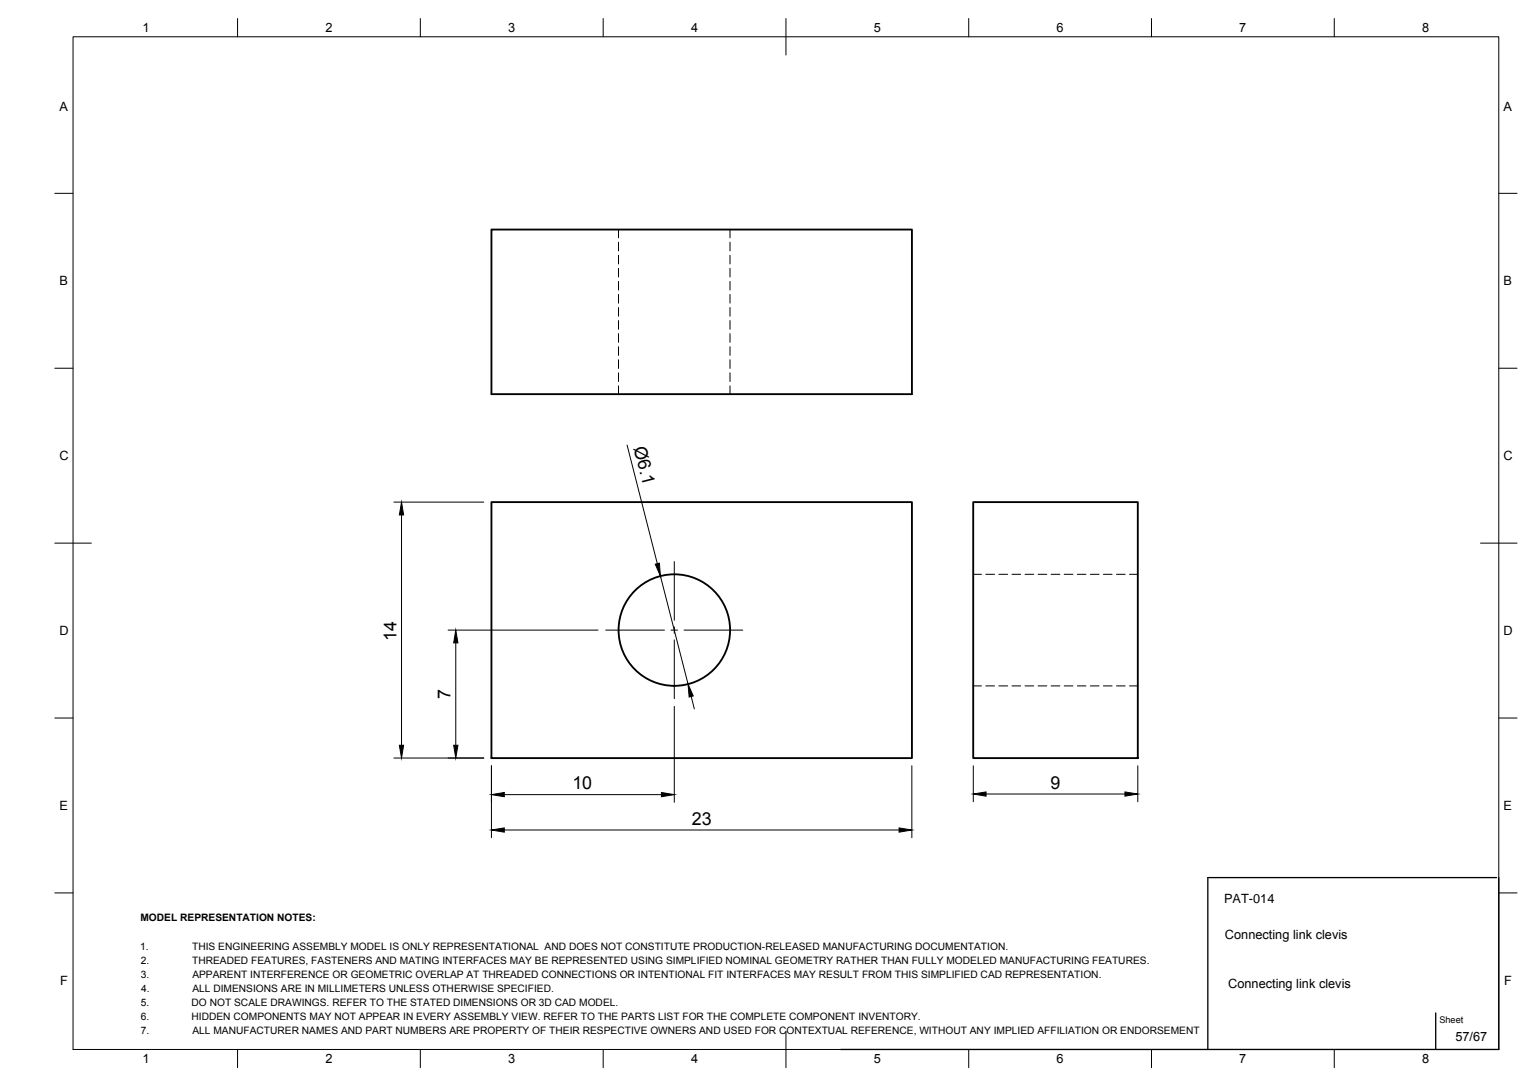
ISO-10303-21;
HEADER;
/* Generated by software containing ST-Developer
 * from STEP Tools, Inc. (www.steptools.com) 
 */

FILE_DESCRIPTION(
/* description */ ('Bin tilter linkage'),
/* implementation_level */ '2;1');

FILE_NAME(
/* name */ 'Connecting link clevis.step',
/* time_stamp */ '2026-10-28T03:26:24-07:00',
/* author */ (''),
/* organization */ (''),
/* preprocessor_version */ 'ST-DEVELOPER v20.2',
/* originating_system */ 'Autodesk Translation Framework v15.17.0.0',
/* authorisation */ '');

FILE_SCHEMA (('AUTOMOTIVE_DESIGN { 1 0 10303 214 3 1 1 }'));
ENDSEC;

DATA;
#10=MECHANICAL_DESIGN_GEOMETRIC_PRESENTATION_REPRESENTATION('',(#963),#23728);
#743=SHAPE_REPRESENTATION_RELATIONSHIP('SRR','None',#24212,#849);
#849=ADVANCED_BREP_SHAPE_REPRESENTATION('',(#1075),#23712);
#963=STYLED_ITEM('',(#24751),#1075);
#1075=MANIFOLD_SOLID_BREP('Body1',#12495);
#1462=FACE_BOUND('',#3732,.T.);
#1463=FACE_BOUND('',#3735,.T.);
#1834=PLANE('',#15279);
#1835=PLANE('',#15280);
#1836=PLANE('',#15281);
#1837=PLANE('',#15282);
#1838=PLANE('',#15283);
#1839=PLANE('',#15284);
#2578=FACE_OUTER_BOUND('',#3730,.T.);
#2579=FACE_OUTER_BOUND('',#3731,.T.);
#2580=FACE_OUTER_BOUND('',#3733,.T.);
#2581=FACE_OUTER_BOUND('',#3734,.T.);
#2582=FACE_OUTER_BOUND('',#3736,.T.);
#2583=FACE_OUTER_BOUND('',#3737,.T.);
#2584=FACE_OUTER_BOUND('',#3738,.T.);
#3730=EDGE_LOOP('',(#10955,#10956,#10957,#10958));
#3731=EDGE_LOOP('',(#10959,#10960,#10961,#10962));
#3732=EDGE_LOOP('',(#10963));
#3733=EDGE_LOOP('',(#10964,#10965,#10966,#10967));
#3734=EDGE_LOOP('',(#10968,#10969,#10970,#10971));
#3735=EDGE_LOOP('',(#10972));
#3736=EDGE_LOOP('',(#10973,#10974,#10975,#10976));
#3737=EDGE_LOOP('',(#10977,#10978,#10979,#10980));
#3738=EDGE_LOOP('',(#10981,#10982,#10983,#10984));
#4437=LINE('',#23111,#5112);
#4438=LINE('',#23116,#5113);
#4439=LINE('',#23118,#5114);
#4440=LINE('',#23120,#5115);
#4441=LINE('',#23121,#5116);
#4442=LINE('',#23124,#5117);
#4443=LINE('',#23126,#5118);
#4444=LINE('',#23127,#5119);
#4445=LINE('',#23130,#5120);
#4446=LINE('',#23132,#5121);
#4447=LINE('',#23133,#5122);
#4448=LINE('',#23135,#5123);
#4449=LINE('',#23136,#5124);
#5112=VECTOR('',#19266,0.305);
#5113=VECTOR('',#19271,1.);
#5114=VECTOR('',#19272,1.);
#5115=VECTOR('',#19273,1.);
#5116=VECTOR('',#19274,1.);
#5117=VECTOR('',#19277,1.);
#5118=VECTOR('',#19278,1.);
#5119=VECTOR('',#19279,1.);
#5120=VECTOR('',#19282,1.);
#5121=VECTOR('',#19283,1.);
#5122=VECTOR('',#19284,1.);
#5123=VECTOR('',#19287,1.);
#5124=VECTOR('',#19288,1.);
#5888=CIRCLE('',#15277,0.305);
#5889=CIRCLE('',#15278,0.305);
#6823=VERTEX_POINT('',#23108);
#6824=VERTEX_POINT('',#23110);
#6825=VERTEX_POINT('',#23114);
#6826=VERTEX_POINT('',#23115);
#6827=VERTEX_POINT('',#23117);
#6828=VERTEX_POINT('',#23119);
#6829=VERTEX_POINT('',#23123);
#6830=VERTEX_POINT('',#23125);
#6831=VERTEX_POINT('',#23129);
#6832=VERTEX_POINT('',#23131);
#8217=EDGE_CURVE('',#6823,#6823,#5888,.T.);
#8218=EDGE_CURVE('',#6823,#6824,#4437,.T.);
#8219=EDGE_CURVE('',#6824,#6824,#5889,.T.);
#8220=EDGE_CURVE('',#6825,#6826,#4438,.T.);
#8221=EDGE_CURVE('',#6826,#6827,#4439,.T.);
#8222=EDGE_CURVE('',#6828,#6827,#4440,.T.);
#8223=EDGE_CURVE('',#6825,#6828,#4441,.T.);
#8224=EDGE_CURVE('',#6829,#6825,#4442,.T.);
#8225=EDGE_CURVE('',#6830,#6828,#4443,.T.);
#8226=EDGE_CURVE('',#6829,#6830,#4444,.T.);
#8227=EDGE_CURVE('',#6831,#6829,#4445,.T.);
#8228=EDGE_CURVE('',#6832,#6830,#4446,.T.);
#8229=EDGE_CURVE('',#6831,#6832,#4447,.T.);
#8230=EDGE_CURVE('',#6826,#6831,#4448,.T.);
#8231=EDGE_CURVE('',#6827,#6832,#4449,.T.);
#10955=ORIENTED_EDGE('',*,*,#8217,.F.);
#10956=ORIENTED_EDGE('',*,*,#8218,.T.);
#10957=ORIENTED_EDGE('',*,*,#8219,.F.);
#10958=ORIENTED_EDGE('',*,*,#8218,.F.);
#10959=ORIENTED_EDGE('',*,*,#8220,.T.);
#10960=ORIENTED_EDGE('',*,*,#8221,.T.);
#10961=ORIENTED_EDGE('',*,*,#8222,.F.);
#10962=ORIENTED_EDGE('',*,*,#8223,.F.);
#10963=ORIENTED_EDGE('',*,*,#8219,.T.);
#10964=ORIENTED_EDGE('',*,*,#8224,.T.);
#10965=ORIENTED_EDGE('',*,*,#8223,.T.);
#10966=ORIENTED_EDGE('',*,*,#8225,.F.);
#10967=ORIENTED_EDGE('',*,*,#8226,.F.);
#10968=ORIENTED_EDGE('',*,*,#8227,.T.);
#10969=ORIENTED_EDGE('',*,*,#8226,.T.);
#10970=ORIENTED_EDGE('',*,*,#8228,.F.);
#10971=ORIENTED_EDGE('',*,*,#8229,.F.);
#10972=ORIENTED_EDGE('',*,*,#8217,.T.);
#10973=ORIENTED_EDGE('',*,*,#8230,.T.);
#10974=ORIENTED_EDGE('',*,*,#8229,.T.);
#10975=ORIENTED_EDGE('',*,*,#8231,.F.);
#10976=ORIENTED_EDGE('',*,*,#8221,.F.);
#10977=ORIENTED_EDGE('',*,*,#8231,.T.);
#10978=ORIENTED_EDGE('',*,*,#8228,.T.);
#10979=ORIENTED_EDGE('',*,*,#8225,.T.);
#10980=ORIENTED_EDGE('',*,*,#8222,.T.);
#10981=ORIENTED_EDGE('',*,*,#8230,.F.);
#10982=ORIENTED_EDGE('',*,*,#8220,.F.);
#10983=ORIENTED_EDGE('',*,*,#8224,.F.);
#10984=ORIENTED_EDGE('',*,*,#8227,.F.);
#11585=CYLINDRICAL_SURFACE('',#15276,0.305);
#12303=ADVANCED_FACE('',(#2578),#11585,.F.);
#12304=ADVANCED_FACE('',(#2579,#1462),#1834,.T.);
#12305=ADVANCED_FACE('',(#2580),#1835,.T.);
#12306=ADVANCED_FACE('',(#2581,#1463),#1836,.T.);
#12307=ADVANCED_FACE('',(#2582),#1837,.T.);
#12308=ADVANCED_FACE('',(#2583),#1838,.T.);
#12309=ADVANCED_FACE('',(#2584),#1839,.F.);
#12495=CLOSED_SHELL('',(#12303,#12304,#12305,#12306,#12307,#12308,#12309));
#15275=AXIS2_PLACEMENT_3D('',#23106,#19260,#19261);
#15276=AXIS2_PLACEMENT_3D('',#23107,#19262,#19263);
#15277=AXIS2_PLACEMENT_3D('',#23109,#19264,#19265);
#15278=AXIS2_PLACEMENT_3D('',#23112,#19267,#19268);
#15279=AXIS2_PLACEMENT_3D('',#23113,#19269,#19270);
#15280=AXIS2_PLACEMENT_3D('',#23122,#19275,#19276);
#15281=AXIS2_PLACEMENT_3D('',#23128,#19280,#19281);
#15282=AXIS2_PLACEMENT_3D('',#23134,#19285,#19286);
#15283=AXIS2_PLACEMENT_3D('',#23137,#19289,#19290);
#15284=AXIS2_PLACEMENT_3D('',#23138,#19291,#19292);
#19260=DIRECTION('axis',(0.,0.,1.));
#19261=DIRECTION('refdir',(1.,0.,0.));
#19262=DIRECTION('center_axis',(0.,1.,0.));
#19263=DIRECTION('ref_axis',(1.,0.,0.));
#19264=DIRECTION('center_axis',(0.,1.,0.));
#19265=DIRECTION('ref_axis',(1.,0.,0.));
#19266=DIRECTION('',(0.,1.,0.));
#19267=DIRECTION('center_axis',(0.,-1.,0.));
#19268=DIRECTION('ref_axis',(1.,0.,0.));
#19269=DIRECTION('center_axis',(0.,1.,0.));
#19270=DIRECTION('ref_axis',(-1.,0.,0.));
#19271=DIRECTION('',(-1.,0.,0.));
#19272=DIRECTION('',(0.,0.,1.));
#19273=DIRECTION('',(-1.,0.,0.));
#19274=DIRECTION('',(0.,0.,1.));
#19275=DIRECTION('center_axis',(1.,0.,0.));
#19276=DIRECTION('ref_axis',(0.,1.,0.));
#19277=DIRECTION('',(0.,1.,0.));
#19278=DIRECTION('',(0.,1.,0.));
#19279=DIRECTION('',(0.,0.,1.));
#19280=DIRECTION('center_axis',(0.,-1.,0.));
#19281=DIRECTION('ref_axis',(1.,0.,0.));
#19282=DIRECTION('',(1.,0.,0.));
#19283=DIRECTION('',(1.,0.,0.));
#19284=DIRECTION('',(0.,0.,1.));
#19285=DIRECTION('center_axis',(-1.,0.,0.));
#19286=DIRECTION('ref_axis',(0.,-1.,0.));
#19287=DIRECTION('',(0.,-1.,0.));
#19288=DIRECTION('',(0.,-1.,0.));
#19289=DIRECTION('center_axis',(0.,0.,1.));
#19290=DIRECTION('ref_axis',(1.,0.,0.));
#19291=DIRECTION('center_axis',(0.,0.,1.));
#19292=DIRECTION('ref_axis',(1.,0.,0.));
#23106=CARTESIAN_POINT('',(0.,0.,0.));
#23107=CARTESIAN_POINT('Origin',(-4.,-4.,11.));
#23108=CARTESIAN_POINT('',(-4.305,-3.9,11.));
#23109=CARTESIAN_POINT('Origin',(-4.,-3.9,11.));
#23110=CARTESIAN_POINT('',(-4.305,-3.,11.));
#23111=CARTESIAN_POINT('',(-4.305,-4.,11.));
#23112=CARTESIAN_POINT('Origin',(-4.,-3.,11.));
#23113=CARTESIAN_POINT('Origin',(-3.3,-3.,9.7));
#23114=CARTESIAN_POINT('',(-3.3,-3.,9.7));
#23115=CARTESIAN_POINT('',(-4.7,-3.,9.7));
#23116=CARTESIAN_POINT('',(-3.3,-3.,9.7));
#23117=CARTESIAN_POINT('',(-4.7,-3.,12.));
#23118=CARTESIAN_POINT('',(-4.7,-3.,9.7));
#23119=CARTESIAN_POINT('',(-3.3,-3.,12.));
#23120=CARTESIAN_POINT('',(-3.3,-3.,12.));
#23121=CARTESIAN_POINT('',(-3.3,-3.,9.7));
#23122=CARTESIAN_POINT('Origin',(-3.3,-3.9,9.7));
#23123=CARTESIAN_POINT('',(-3.3,-3.9,9.7));
#23124=CARTESIAN_POINT('',(-3.3,-3.9,9.7));
#23125=CARTESIAN_POINT('',(-3.3,-3.9,12.));
#23126=CARTESIAN_POINT('',(-3.3,-3.9,12.));
#23127=CARTESIAN_POINT('',(-3.3,-3.9,9.7));
#23128=CARTESIAN_POINT('Origin',(-4.7,-3.9,9.7));
#23129=CARTESIAN_POINT('',(-4.7,-3.9,9.7));
#23130=CARTESIAN_POINT('',(-4.7,-3.9,9.7));
#23131=CARTESIAN_POINT('',(-4.7,-3.9,12.));
#23132=CARTESIAN_POINT('',(-4.7,-3.9,12.));
#23133=CARTESIAN_POINT('',(-4.7,-3.9,9.7));
#23134=CARTESIAN_POINT('Origin',(-4.7,-3.,9.7));
#23135=CARTESIAN_POINT('',(-4.7,-3.,9.7));
#23136=CARTESIAN_POINT('',(-4.7,-3.,12.));
#23137=CARTESIAN_POINT('Origin',(-4.,-3.45,12.));
#23138=CARTESIAN_POINT('Origin',(-4.,-3.45,9.7));
#23595=UNCERTAINTY_MEASURE_WITH_UNIT(LENGTH_MEASURE(0.001),#23729,
'DISTANCE_ACCURACY_VALUE',
'Maximum model space distance between geometric entities at asserted c
onnectivities');
#23611=UNCERTAINTY_MEASURE_WITH_UNIT(LENGTH_MEASURE(0.001),#23729,
'DISTANCE_ACCURACY_VALUE',
'Maximum model space distance between geometric entities at asserted c
onnectivities');
#23712=(
GEOMETRIC_REPRESENTATION_CONTEXT(3)
GLOBAL_UNCERTAINTY_ASSIGNED_CONTEXT((#23595))
GLOBAL_UNIT_ASSIGNED_CONTEXT((#23729,#23731,#23732))
REPRESENTATION_CONTEXT('','3D')
);
#23728=(
GEOMETRIC_REPRESENTATION_CONTEXT(3)
GLOBAL_UNCERTAINTY_ASSIGNED_CONTEXT((#23611))
GLOBAL_UNIT_ASSIGNED_CONTEXT((#23729,#23731,#23732))
REPRESENTATION_CONTEXT('','3D')
);
#23729=(
LENGTH_UNIT()
NAMED_UNIT(*)
SI_UNIT(.CENTI.,.METRE.)
);
#23731=(
NAMED_UNIT(*)
PLANE_ANGLE_UNIT()
SI_UNIT($,.RADIAN.)
);
#23732=(
NAMED_UNIT(*)
SI_UNIT($,.STERADIAN.)
SOLID_ANGLE_UNIT()
);
#23833=SHAPE_DEFINITION_REPRESENTATION(#24071,#24212);
#24071=PRODUCT_DEFINITION_SHAPE('',$,#24329);
#24212=SHAPE_REPRESENTATION('',(#15275),#23712);
#24228=PRODUCT_DEFINITION_CONTEXT('part definition',#24578,'design');
#24329=PRODUCT_DEFINITION('Connecting link clevis',
'Connecting link clevis',#24445,#24228);
#24445=PRODUCT_DEFINITION_FORMATION('',$,#24680);
#24578=APPLICATION_CONTEXT(
'Core Data for Automotive Mechanical Design Process');
#24579=PRODUCT_CONTEXT('part definition',#24578,'mechanical');
#24680=PRODUCT('Connecting link clevis','Connecting link clevis',
'Connecting link clevis',(#24579));
#24745=COLOUR_RGB('Light Blue',0.38,0.62,0.78);
#24746=FILL_AREA_STYLE_COLOUR('',#24745);
#24747=FILL_AREA_STYLE('',(#24746));
#24748=SURFACE_STYLE_FILL_AREA(#24747);
#24749=SURFACE_SIDE_STYLE('',(#24748));
#24750=SURFACE_STYLE_USAGE(.BOTH.,#24749);
#24751=PRESENTATION_STYLE_ASSIGNMENT((#24750));
ENDSEC;
END-ISO-10303-21;
